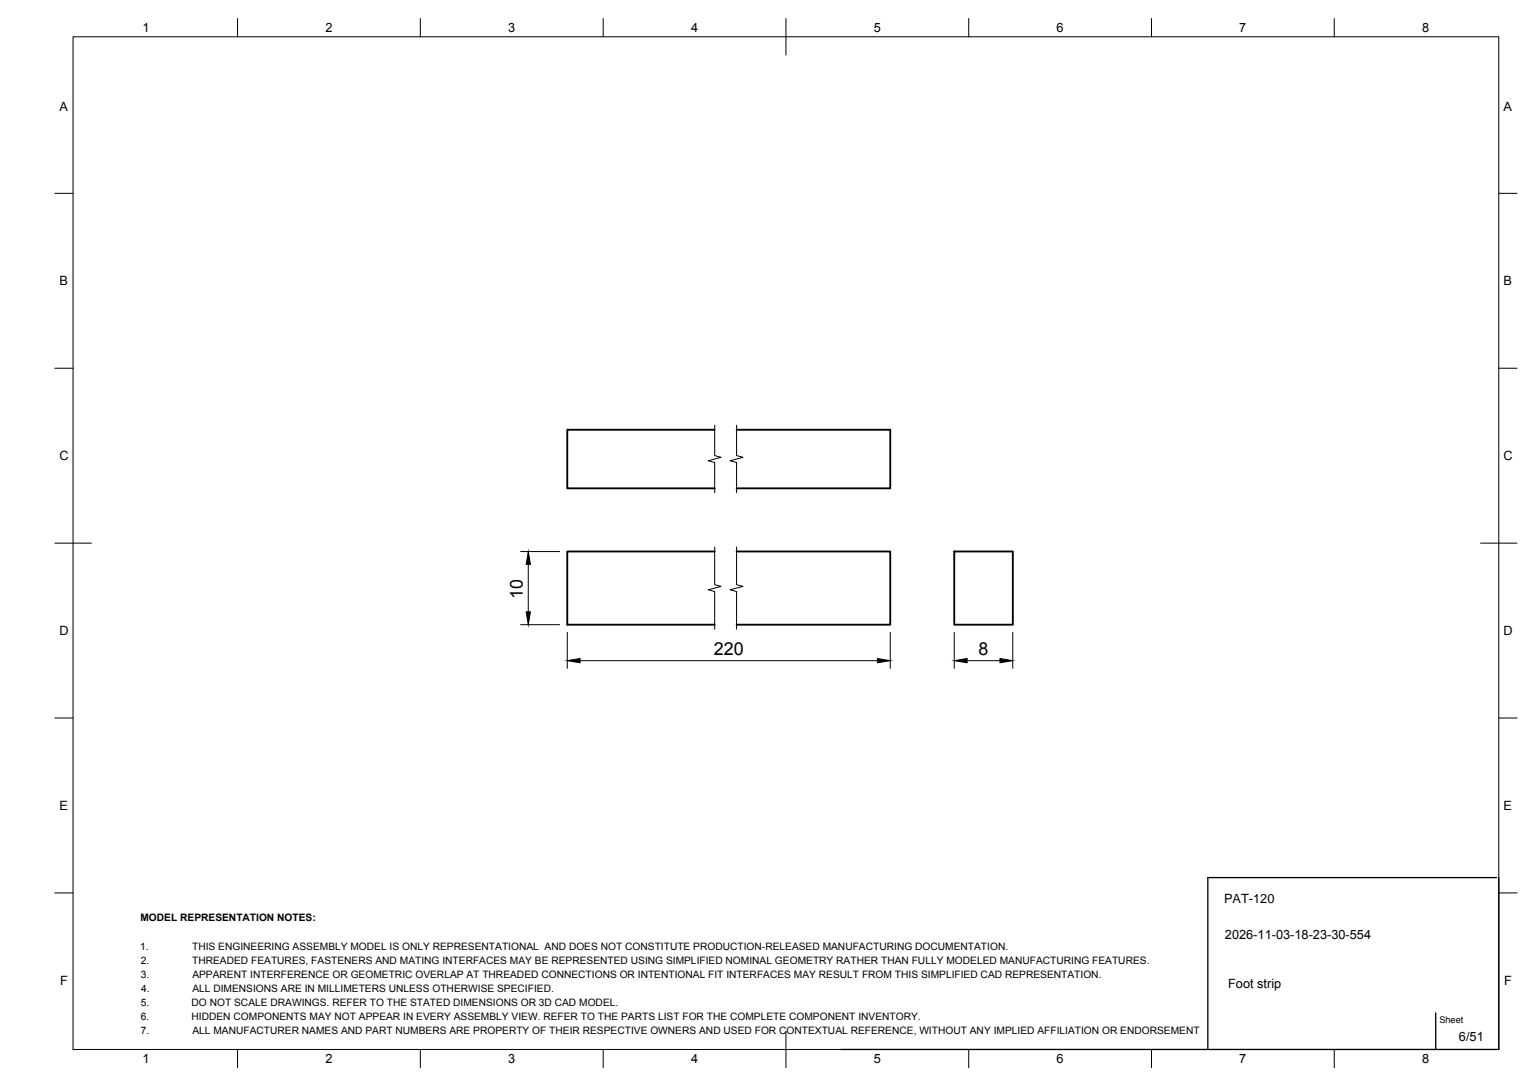
ISO-10303-21;
HEADER;
/* Generated by software containing ST-Developer
 * from STEP Tools, Inc. (www.steptools.com) 
 */

FILE_DESCRIPTION(
/* description */ ('Vibration shaker table dummy'),
/* implementation_level */ '2;1');

FILE_NAME(
/* name */ 'Foot strip.step',
/* time_stamp */ '2026-10-27T10:55:14-07:00',
/* author */ (''),
/* organization */ (''),
/* preprocessor_version */ 'ST-DEVELOPER v20.2',
/* originating_system */ 'Autodesk Translation Framework v15.17.0.0',
/* authorisation */ '');

FILE_SCHEMA (('AUTOMOTIVE_DESIGN { 1 0 10303 214 3 1 1 }'));
ENDSEC;

DATA;
#10=MECHANICAL_DESIGN_GEOMETRIC_PRESENTATION_REPRESENTATION('',(#687),#22394);
#595=SHAPE_REPRESENTATION_RELATIONSHIP('SRR','None',#22641,#641);
#641=ADVANCED_BREP_SHAPE_REPRESENTATION('',(#733),#22347);
#687=STYLED_ITEM('',(#22947),#733);
#733=MANIFOLD_SOLID_BREP('Body1',#9205);
#1066=PLANE('',#9836);
#1067=PLANE('',#9837);
#1068=PLANE('',#9838);
#1069=PLANE('',#9839);
#1070=PLANE('',#9840);
#1071=PLANE('',#9841);
#1369=FACE_OUTER_BOUND('',#1911,.T.);
#1370=FACE_OUTER_BOUND('',#1912,.T.);
#1371=FACE_OUTER_BOUND('',#1913,.T.);
#1372=FACE_OUTER_BOUND('',#1914,.T.);
#1373=FACE_OUTER_BOUND('',#1915,.T.);
#1374=FACE_OUTER_BOUND('',#1916,.T.);
#1911=EDGE_LOOP('',(#6402,#6403,#6404,#6405));
#1912=EDGE_LOOP('',(#6406,#6407,#6408,#6409));
#1913=EDGE_LOOP('',(#6410,#6411,#6412,#6413));
#1914=EDGE_LOOP('',(#6414,#6415,#6416,#6417));
#1915=EDGE_LOOP('',(#6418,#6419,#6420,#6421));
#1916=EDGE_LOOP('',(#6422,#6423,#6424,#6425));
#2656=LINE('',#14114,#3275);
#2657=LINE('',#14116,#3276);
#2658=LINE('',#14118,#3277);
#2659=LINE('',#14119,#3278);
#2660=LINE('',#14122,#3279);
#2661=LINE('',#14124,#3280);
#2662=LINE('',#14125,#3281);
#2663=LINE('',#14128,#3282);
#2664=LINE('',#14130,#3283);
#2665=LINE('',#14131,#3284);
#2666=LINE('',#14133,#3285);
#2667=LINE('',#14134,#3286);
#3275=VECTOR('',#11138,1.);
#3276=VECTOR('',#11139,1.);
#3277=VECTOR('',#11140,1.);
#3278=VECTOR('',#11141,1.);
#3279=VECTOR('',#11144,1.);
#3280=VECTOR('',#11145,1.);
#3281=VECTOR('',#11146,1.);
#3282=VECTOR('',#11149,1.);
#3283=VECTOR('',#11150,1.);
#3284=VECTOR('',#11151,1.);
#3285=VECTOR('',#11154,1.);
#3286=VECTOR('',#11155,1.);
#4419=VERTEX_POINT('',#14112);
#4420=VERTEX_POINT('',#14113);
#4421=VERTEX_POINT('',#14115);
#4422=VERTEX_POINT('',#14117);
#4423=VERTEX_POINT('',#14121);
#4424=VERTEX_POINT('',#14123);
#4425=VERTEX_POINT('',#14127);
#4426=VERTEX_POINT('',#14129);
#5194=EDGE_CURVE('',#4419,#4420,#2656,.T.);
#5195=EDGE_CURVE('',#4420,#4421,#2657,.T.);
#5196=EDGE_CURVE('',#4422,#4421,#2658,.T.);
#5197=EDGE_CURVE('',#4419,#4422,#2659,.T.);
#5198=EDGE_CURVE('',#4423,#4419,#2660,.T.);
#5199=EDGE_CURVE('',#4424,#4422,#2661,.T.);
#5200=EDGE_CURVE('',#4423,#4424,#2662,.T.);
#5201=EDGE_CURVE('',#4425,#4423,#2663,.T.);
#5202=EDGE_CURVE('',#4426,#4424,#2664,.T.);
#5203=EDGE_CURVE('',#4425,#4426,#2665,.T.);
#5204=EDGE_CURVE('',#4420,#4425,#2666,.T.);
#5205=EDGE_CURVE('',#4421,#4426,#2667,.T.);
#6402=ORIENTED_EDGE('',*,*,#5194,.T.);
#6403=ORIENTED_EDGE('',*,*,#5195,.T.);
#6404=ORIENTED_EDGE('',*,*,#5196,.F.);
#6405=ORIENTED_EDGE('',*,*,#5197,.F.);
#6406=ORIENTED_EDGE('',*,*,#5198,.T.);
#6407=ORIENTED_EDGE('',*,*,#5197,.T.);
#6408=ORIENTED_EDGE('',*,*,#5199,.F.);
#6409=ORIENTED_EDGE('',*,*,#5200,.F.);
#6410=ORIENTED_EDGE('',*,*,#5201,.T.);
#6411=ORIENTED_EDGE('',*,*,#5200,.T.);
#6412=ORIENTED_EDGE('',*,*,#5202,.F.);
#6413=ORIENTED_EDGE('',*,*,#5203,.F.);
#6414=ORIENTED_EDGE('',*,*,#5204,.T.);
#6415=ORIENTED_EDGE('',*,*,#5203,.T.);
#6416=ORIENTED_EDGE('',*,*,#5205,.F.);
#6417=ORIENTED_EDGE('',*,*,#5195,.F.);
#6418=ORIENTED_EDGE('',*,*,#5205,.T.);
#6419=ORIENTED_EDGE('',*,*,#5202,.T.);
#6420=ORIENTED_EDGE('',*,*,#5199,.T.);
#6421=ORIENTED_EDGE('',*,*,#5196,.T.);
#6422=ORIENTED_EDGE('',*,*,#5204,.F.);
#6423=ORIENTED_EDGE('',*,*,#5194,.F.);
#6424=ORIENTED_EDGE('',*,*,#5198,.F.);
#6425=ORIENTED_EDGE('',*,*,#5201,.F.);
#8734=ADVANCED_FACE('',(#1369),#1066,.T.);
#8735=ADVANCED_FACE('',(#1370),#1067,.T.);
#8736=ADVANCED_FACE('',(#1371),#1068,.T.);
#8737=ADVANCED_FACE('',(#1372),#1069,.T.);
#8738=ADVANCED_FACE('',(#1373),#1070,.T.);
#8739=ADVANCED_FACE('',(#1374),#1071,.F.);
#9205=CLOSED_SHELL('',(#8734,#8735,#8736,#8737,#8738,#8739));
#9835=AXIS2_PLACEMENT_3D('',#14110,#11134,#11135);
#9836=AXIS2_PLACEMENT_3D('',#14111,#11136,#11137);
#9837=AXIS2_PLACEMENT_3D('',#14120,#11142,#11143);
#9838=AXIS2_PLACEMENT_3D('',#14126,#11147,#11148);
#9839=AXIS2_PLACEMENT_3D('',#14132,#11152,#11153);
#9840=AXIS2_PLACEMENT_3D('',#14135,#11156,#11157);
#9841=AXIS2_PLACEMENT_3D('',#14136,#11158,#11159);
#11134=DIRECTION('axis',(0.,0.,1.));
#11135=DIRECTION('refdir',(1.,0.,0.));
#11136=DIRECTION('center_axis',(0.,1.,0.));
#11137=DIRECTION('ref_axis',(-1.,0.,0.));
#11138=DIRECTION('',(-1.,0.,0.));
#11139=DIRECTION('',(0.,0.,1.));
#11140=DIRECTION('',(-1.,0.,0.));
#11141=DIRECTION('',(0.,0.,1.));
#11142=DIRECTION('center_axis',(1.,0.,0.));
#11143=DIRECTION('ref_axis',(0.,1.,0.));
#11144=DIRECTION('',(0.,1.,0.));
#11145=DIRECTION('',(0.,1.,0.));
#11146=DIRECTION('',(0.,0.,1.));
#11147=DIRECTION('center_axis',(0.,-1.,0.));
#11148=DIRECTION('ref_axis',(1.,0.,0.));
#11149=DIRECTION('',(1.,0.,0.));
#11150=DIRECTION('',(1.,0.,0.));
#11151=DIRECTION('',(0.,0.,1.));
#11152=DIRECTION('center_axis',(-1.,0.,0.));
#11153=DIRECTION('ref_axis',(0.,-1.,0.));
#11154=DIRECTION('',(0.,-1.,0.));
#11155=DIRECTION('',(0.,-1.,0.));
#11156=DIRECTION('center_axis',(0.,0.,1.));
#11157=DIRECTION('ref_axis',(1.,0.,0.));
#11158=DIRECTION('center_axis',(0.,0.,1.));
#11159=DIRECTION('ref_axis',(1.,0.,0.));
#14110=CARTESIAN_POINT('',(0.,0.,0.));
#14111=CARTESIAN_POINT('Origin',(11.,-7.2,-2.2));
#14112=CARTESIAN_POINT('',(11.,-7.2,-2.2));
#14113=CARTESIAN_POINT('',(-11.,-7.2,-2.2));
#14114=CARTESIAN_POINT('',(11.,-7.2,-2.2));
#14115=CARTESIAN_POINT('',(-11.,-7.2,-1.2));
#14116=CARTESIAN_POINT('',(-11.,-7.2,-2.2));
#14117=CARTESIAN_POINT('',(11.,-7.2,-1.2));
#14118=CARTESIAN_POINT('',(11.,-7.2,-1.2));
#14119=CARTESIAN_POINT('',(11.,-7.2,-2.2));
#14120=CARTESIAN_POINT('Origin',(11.,-8.,-2.2));
#14121=CARTESIAN_POINT('',(11.,-8.,-2.2));
#14122=CARTESIAN_POINT('',(11.,-8.,-2.2));
#14123=CARTESIAN_POINT('',(11.,-8.,-1.2));
#14124=CARTESIAN_POINT('',(11.,-8.,-1.2));
#14125=CARTESIAN_POINT('',(11.,-8.,-2.2));
#14126=CARTESIAN_POINT('Origin',(-11.,-8.,-2.2));
#14127=CARTESIAN_POINT('',(-11.,-8.,-2.2));
#14128=CARTESIAN_POINT('',(-11.,-8.,-2.2));
#14129=CARTESIAN_POINT('',(-11.,-8.,-1.2));
#14130=CARTESIAN_POINT('',(-11.,-8.,-1.2));
#14131=CARTESIAN_POINT('',(-11.,-8.,-2.2));
#14132=CARTESIAN_POINT('Origin',(-11.,-7.2,-2.2));
#14133=CARTESIAN_POINT('',(-11.,-7.2,-2.2));
#14134=CARTESIAN_POINT('',(-11.,-7.2,-1.2));
#14135=CARTESIAN_POINT('Origin',(0.,-7.6,-1.2));
#14136=CARTESIAN_POINT('Origin',(0.,-7.6,-2.2));
#22296=UNCERTAINTY_MEASURE_WITH_UNIT(LENGTH_MEASURE(0.001),#22395,
'DISTANCE_ACCURACY_VALUE',
'Maximum model space distance between geometric entities at asserted c
onnectivities');
#22343=UNCERTAINTY_MEASURE_WITH_UNIT(LENGTH_MEASURE(0.001),#22395,
'DISTANCE_ACCURACY_VALUE',
'Maximum model space distance between geometric entities at asserted c
onnectivities');
#22347=(
GEOMETRIC_REPRESENTATION_CONTEXT(3)
GLOBAL_UNCERTAINTY_ASSIGNED_CONTEXT((#22296))
GLOBAL_UNIT_ASSIGNED_CONTEXT((#22395,#22397,#22398))
REPRESENTATION_CONTEXT('','3D')
);
#22394=(
GEOMETRIC_REPRESENTATION_CONTEXT(3)
GLOBAL_UNCERTAINTY_ASSIGNED_CONTEXT((#22343))
GLOBAL_UNIT_ASSIGNED_CONTEXT((#22395,#22397,#22398))
REPRESENTATION_CONTEXT('','3D')
);
#22395=(
LENGTH_UNIT()
NAMED_UNIT(*)
SI_UNIT(.CENTI.,.METRE.)
);
#22397=(
NAMED_UNIT(*)
PLANE_ANGLE_UNIT()
SI_UNIT($,.RADIAN.)
);
#22398=(
NAMED_UNIT(*)
SI_UNIT($,.STERADIAN.)
SOLID_ANGLE_UNIT()
);
#22402=SHAPE_DEFINITION_REPRESENTATION(#22452,#22641);
#22452=PRODUCT_DEFINITION_SHAPE('',$,#22692);
#22641=SHAPE_REPRESENTATION('',(#9835),#22347);
#22688=PRODUCT_DEFINITION_CONTEXT('part definition',#22840,'design');
#22692=PRODUCT_DEFINITION('Foot strip','Foot strip',#22742,#22688);
#22742=PRODUCT_DEFINITION_FORMATION('',$,#22845);
#22840=APPLICATION_CONTEXT(
'Core Data for Automotive Mechanical Design Process');
#22841=PRODUCT_CONTEXT('part definition',#22840,'mechanical');
#22845=PRODUCT('Foot strip','Foot strip','Foot strip',(#22841));
#22941=COLOUR_RGB('Light Blue',0.38,0.62,0.78);
#22942=FILL_AREA_STYLE_COLOUR('',#22941);
#22943=FILL_AREA_STYLE('',(#22942));
#22944=SURFACE_STYLE_FILL_AREA(#22943);
#22945=SURFACE_SIDE_STYLE('',(#22944));
#22946=SURFACE_STYLE_USAGE(.BOTH.,#22945);
#22947=PRESENTATION_STYLE_ASSIGNMENT((#22946));
ENDSEC;
END-ISO-10303-21;
